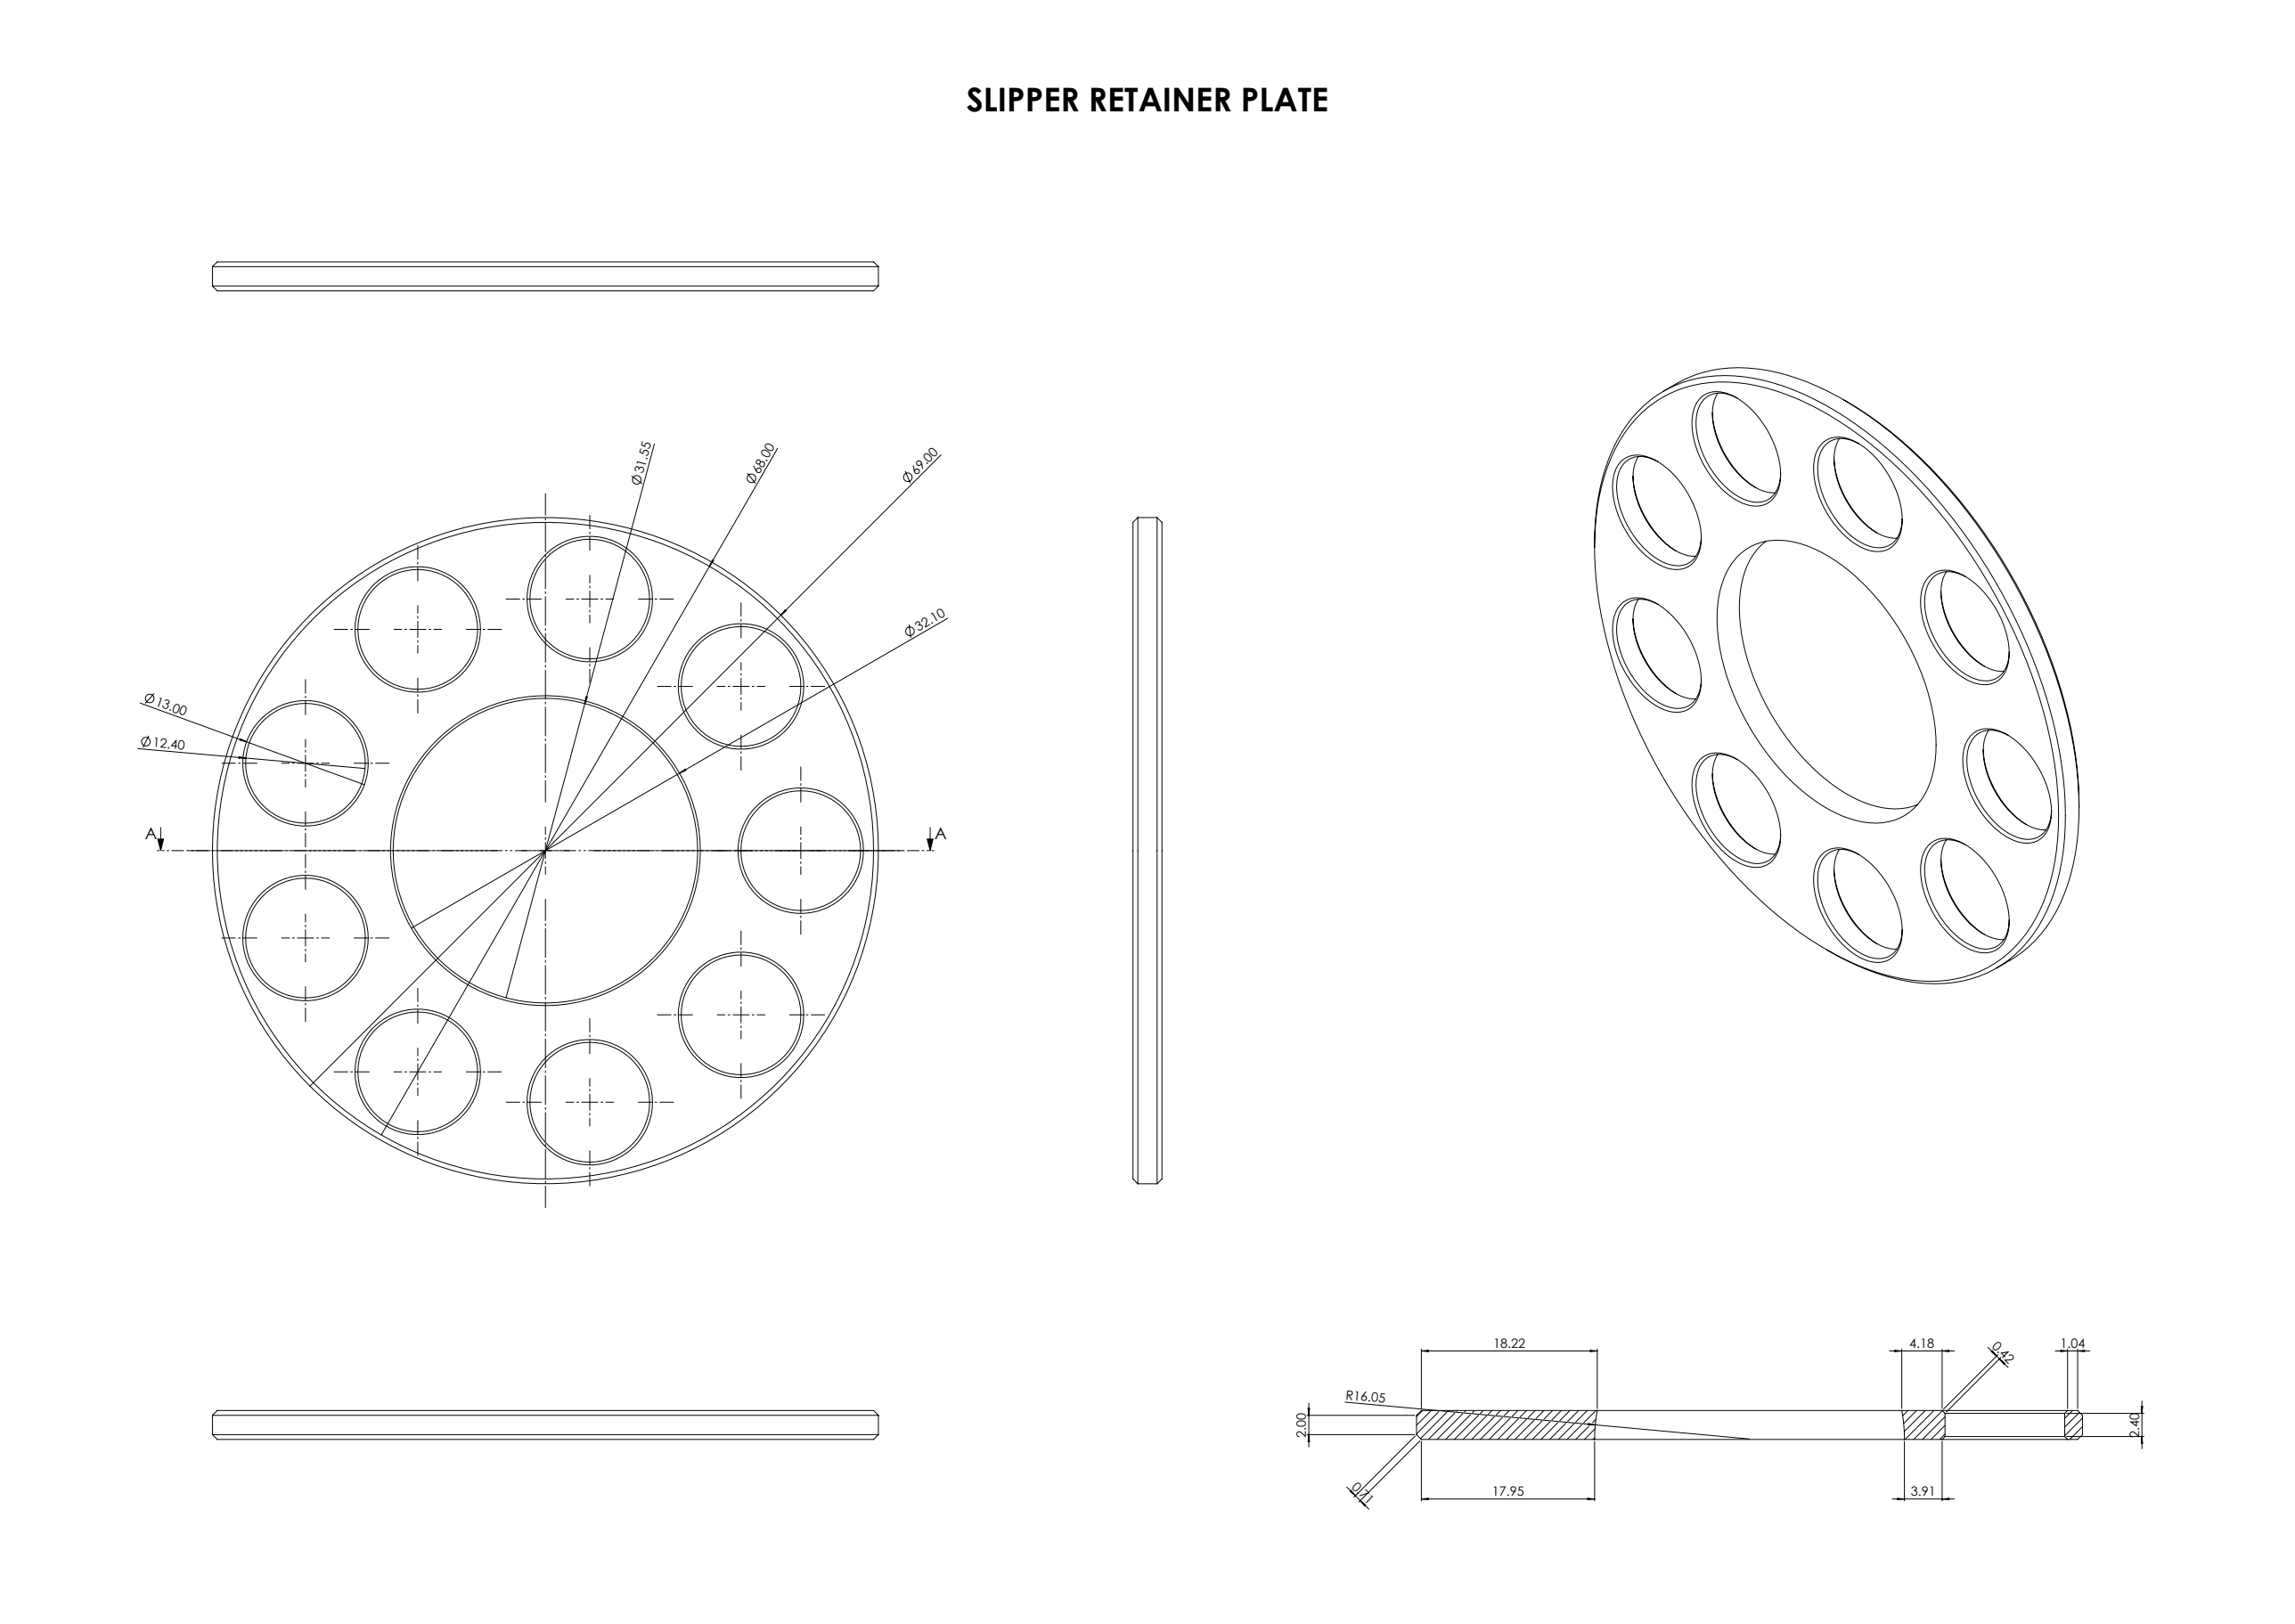
ISO-10303-21;
HEADER;
/* Generated by software containing ST-Developer
 * from STEP Tools, Inc. (www.steptools.com) 
 */

FILE_DESCRIPTION(
/* description */ (''),
/* implementation_level */ '2;1');

FILE_NAME(
/* name */ '08_Slipper_Retainer_Plate.step',
/* time_stamp */ '2026-10-23T00:52:27+05:00',
/* author */ (''),
/* organization */ (''),
/* preprocessor_version */ 'ST-DEVELOPER v20.2',
/* originating_system */ 'Autodesk Translation Framework v15.15.0.0',
/* authorisation */ '');

FILE_SCHEMA (('AUTOMOTIVE_DESIGN { 1 0 10303 214 3 1 1 }'));
ENDSEC;

DATA;
#10=MECHANICAL_DESIGN_GEOMETRIC_PRESENTATION_REPRESENTATION('',(#1548),#59204);
#1508=SHAPE_REPRESENTATION_RELATIONSHIP('SRR','None',#59297,#1528);
#1528=ADVANCED_BREP_SHAPE_REPRESENTATION('',(#1575),#59184);
#1548=STYLED_ITEM('',(#59579),#1575);
#1575=MANIFOLD_SOLID_BREP('Retainer plate',#22804);
#1595=SPHERICAL_SURFACE('',#23116,1.605);
#1599=FACE_BOUND('',#3977,.T.);
#1600=FACE_BOUND('',#3978,.T.);
#1601=FACE_BOUND('',#3979,.T.);
#1602=FACE_BOUND('',#3980,.T.);
#1603=FACE_BOUND('',#3981,.T.);
#1604=FACE_BOUND('',#3982,.T.);
#1605=FACE_BOUND('',#3983,.T.);
#1606=FACE_BOUND('',#3984,.T.);
#1607=FACE_BOUND('',#3985,.T.);
#1608=FACE_BOUND('',#3986,.T.);
#1609=FACE_BOUND('',#3989,.T.);
#1610=FACE_BOUND('',#3990,.T.);
#1611=FACE_BOUND('',#3991,.T.);
#1612=FACE_BOUND('',#3992,.T.);
#1613=FACE_BOUND('',#3993,.T.);
#1614=FACE_BOUND('',#3994,.T.);
#1615=FACE_BOUND('',#3995,.T.);
#1616=FACE_BOUND('',#3996,.T.);
#1617=FACE_BOUND('',#3997,.T.);
#1618=FACE_BOUND('',#3998,.T.);
#1810=PLANE('',#23052);
#1811=PLANE('',#23065);
#2409=CYLINDRICAL_SURFACE('',#23050,0.62);
#2410=CYLINDRICAL_SURFACE('',#23078,0.62);
#2411=CYLINDRICAL_SURFACE('',#23083,0.62);
#2412=CYLINDRICAL_SURFACE('',#23088,0.62);
#2413=CYLINDRICAL_SURFACE('',#23093,0.62);
#2414=CYLINDRICAL_SURFACE('',#23098,0.62);
#2415=CYLINDRICAL_SURFACE('',#23103,0.62);
#2416=CYLINDRICAL_SURFACE('',#23108,0.62);
#2417=CYLINDRICAL_SURFACE('',#23113,0.62);
#2418=CYLINDRICAL_SURFACE('',#23120,3.45);
#2669=FACE_OUTER_BOUND('',#3974,.T.);
#2670=FACE_OUTER_BOUND('',#3975,.T.);
#2671=FACE_OUTER_BOUND('',#3976,.T.);
#2672=FACE_OUTER_BOUND('',#3987,.T.);
#2673=FACE_OUTER_BOUND('',#3988,.T.);
#2674=FACE_OUTER_BOUND('',#3999,.T.);
#2675=FACE_OUTER_BOUND('',#4000,.T.);
#2676=FACE_OUTER_BOUND('',#4001,.T.);
#2677=FACE_OUTER_BOUND('',#4002,.T.);
#2678=FACE_OUTER_BOUND('',#4003,.T.);
#2679=FACE_OUTER_BOUND('',#4004,.T.);
#2680=FACE_OUTER_BOUND('',#4005,.T.);
#2681=FACE_OUTER_BOUND('',#4006,.T.);
#2682=FACE_OUTER_BOUND('',#4007,.T.);
#2683=FACE_OUTER_BOUND('',#4008,.T.);
#2684=FACE_OUTER_BOUND('',#4009,.T.);
#2685=FACE_OUTER_BOUND('',#4010,.T.);
#2686=FACE_OUTER_BOUND('',#4011,.T.);
#2687=FACE_OUTER_BOUND('',#4012,.T.);
#2688=FACE_OUTER_BOUND('',#4013,.T.);
#2689=FACE_OUTER_BOUND('',#4014,.T.);
#2690=FACE_OUTER_BOUND('',#4015,.T.);
#2691=FACE_OUTER_BOUND('',#4016,.T.);
#2692=FACE_OUTER_BOUND('',#4017,.T.);
#2693=FACE_OUTER_BOUND('',#4018,.T.);
#2694=FACE_OUTER_BOUND('',#4019,.T.);
#2695=FACE_OUTER_BOUND('',#4020,.T.);
#2696=FACE_OUTER_BOUND('',#4021,.T.);
#2697=FACE_OUTER_BOUND('',#4022,.T.);
#2698=FACE_OUTER_BOUND('',#4023,.T.);
#2699=FACE_OUTER_BOUND('',#4024,.T.);
#2700=FACE_OUTER_BOUND('',#4025,.T.);
#2701=FACE_OUTER_BOUND('',#4026,.T.);
#3974=EDGE_LOOP('',(#14662,#14663,#14664,#14665));
#3975=EDGE_LOOP('',(#14666,#14667,#14668,#14669));
#3976=EDGE_LOOP('',(#14670));
#3977=EDGE_LOOP('',(#14671));
#3978=EDGE_LOOP('',(#14672));
#3979=EDGE_LOOP('',(#14673));
#3980=EDGE_LOOP('',(#14674));
#3981=EDGE_LOOP('',(#14675));
#3982=EDGE_LOOP('',(#14676));
#3983=EDGE_LOOP('',(#14677));
#3984=EDGE_LOOP('',(#14678));
#3985=EDGE_LOOP('',(#14679));
#3986=EDGE_LOOP('',(#14680));
#3987=EDGE_LOOP('',(#14681,#14682,#14683,#14684));
#3988=EDGE_LOOP('',(#14685));
#3989=EDGE_LOOP('',(#14686));
#3990=EDGE_LOOP('',(#14687));
#3991=EDGE_LOOP('',(#14688));
#3992=EDGE_LOOP('',(#14689));
#3993=EDGE_LOOP('',(#14690));
#3994=EDGE_LOOP('',(#14691));
#3995=EDGE_LOOP('',(#14692));
#3996=EDGE_LOOP('',(#14693));
#3997=EDGE_LOOP('',(#14694));
#3998=EDGE_LOOP('',(#14695));
#3999=EDGE_LOOP('',(#14696,#14697,#14698,#14699));
#4000=EDGE_LOOP('',(#14700,#14701,#14702,#14703));
#4001=EDGE_LOOP('',(#14704,#14705,#14706,#14707));
#4002=EDGE_LOOP('',(#14708,#14709,#14710,#14711));
#4003=EDGE_LOOP('',(#14712,#14713,#14714,#14715));
#4004=EDGE_LOOP('',(#14716,#14717,#14718,#14719));
#4005=EDGE_LOOP('',(#14720,#14721,#14722,#14723));
#4006=EDGE_LOOP('',(#14724,#14725,#14726,#14727));
#4007=EDGE_LOOP('',(#14728,#14729,#14730,#14731));
#4008=EDGE_LOOP('',(#14732,#14733,#14734,#14735));
#4009=EDGE_LOOP('',(#14736,#14737,#14738,#14739));
#4010=EDGE_LOOP('',(#14740,#14741,#14742,#14743));
#4011=EDGE_LOOP('',(#14744,#14745,#14746,#14747));
#4012=EDGE_LOOP('',(#14748,#14749,#14750,#14751));
#4013=EDGE_LOOP('',(#14752,#14753,#14754,#14755));
#4014=EDGE_LOOP('',(#14756,#14757,#14758,#14759));
#4015=EDGE_LOOP('',(#14760,#14761,#14762,#14763));
#4016=EDGE_LOOP('',(#14764,#14765,#14766,#14767));
#4017=EDGE_LOOP('',(#14768,#14769,#14770,#14771));
#4018=EDGE_LOOP('',(#14772,#14773,#14774,#14775));
#4019=EDGE_LOOP('',(#14776,#14777,#14778,#14779));
#4020=EDGE_LOOP('',(#14780,#14781,#14782,#14783));
#4021=EDGE_LOOP('',(#14784,#14785,#14786,#14787));
#4022=EDGE_LOOP('',(#14788,#14789,#14790,#14791));
#4023=EDGE_LOOP('',(#14792,#14793,#14794,#14795));
#4024=EDGE_LOOP('',(#14796,#14797,#14798,#14799));
#4025=EDGE_LOOP('',(#14800,#14801,#14802,#14803));
#4026=EDGE_LOOP('',(#14804,#14805,#14806,#14807));
#5490=LINE('',#30697,#6923);
#5491=LINE('',#30701,#6924);
#5492=LINE('',#30727,#6925);
#5493=LINE('',#30751,#6926);
#5494=LINE('',#30755,#6927);
#5495=LINE('',#30758,#6928);
#5496=LINE('',#30761,#6929);
#5497=LINE('',#30765,#6930);
#5498=LINE('',#30768,#6931);
#5499=LINE('',#30771,#6932);
#5500=LINE('',#30775,#6933);
#5501=LINE('',#30778,#6934);
#5502=LINE('',#30781,#6935);
#5503=LINE('',#30785,#6936);
#5504=LINE('',#30788,#6937);
#5505=LINE('',#30791,#6938);
#5506=LINE('',#30795,#6939);
#5507=LINE('',#30798,#6940);
#5508=LINE('',#30801,#6941);
#5509=LINE('',#30805,#6942);
#5510=LINE('',#30808,#6943);
#5511=LINE('',#30811,#6944);
#5512=LINE('',#30815,#6945);
#5513=LINE('',#30818,#6946);
#5514=LINE('',#30821,#6947);
#5515=LINE('',#30825,#6948);
#5516=LINE('',#30828,#6949);
#5517=LINE('',#30834,#6950);
#5518=LINE('',#30838,#6951);
#5519=LINE('',#30840,#6952);
#6923=VECTOR('',#25124,0.635);
#6924=VECTOR('',#25129,0.62);
#6925=VECTOR('',#25158,0.635);
#6926=VECTOR('',#25183,0.635);
#6927=VECTOR('',#25188,0.62);
#6928=VECTOR('',#25193,0.635);
#6929=VECTOR('',#25196,0.635);
#6930=VECTOR('',#25201,0.62);
#6931=VECTOR('',#25206,0.635);
#6932=VECTOR('',#25209,0.635);
#6933=VECTOR('',#25214,0.62);
#6934=VECTOR('',#25219,0.635);
#6935=VECTOR('',#25222,0.635);
#6936=VECTOR('',#25227,0.62);
#6937=VECTOR('',#25232,0.635);
#6938=VECTOR('',#25235,0.635);
#6939=VECTOR('',#25240,0.62);
#6940=VECTOR('',#25245,0.635);
#6941=VECTOR('',#25248,0.635);
#6942=VECTOR('',#25253,0.62);
#6943=VECTOR('',#25258,0.635);
#6944=VECTOR('',#25261,0.635);
#6945=VECTOR('',#25266,0.62);
#6946=VECTOR('',#25271,0.635);
#6947=VECTOR('',#25274,0.635);
#6948=VECTOR('',#25279,0.62);
#6949=VECTOR('',#25284,0.635);
#6950=VECTOR('',#25293,3.425);
#6951=VECTOR('',#25298,3.45);
#6952=VECTOR('',#25301,3.425);
#8356=CIRCLE('',#23048,0.65);
#8357=CIRCLE('',#23049,0.62);
#8358=CIRCLE('',#23051,0.62);
#8359=CIRCLE('',#23053,3.4);
#8360=CIRCLE('',#23054,0.65);
#8361=CIRCLE('',#23055,0.65);
#8362=CIRCLE('',#23056,0.65);
#8363=CIRCLE('',#23057,0.65);
#8364=CIRCLE('',#23058,1.57765648986083);
#8365=CIRCLE('',#23059,0.65);
#8366=CIRCLE('',#23060,0.65);
#8367=CIRCLE('',#23061,0.65);
#8368=CIRCLE('',#23062,0.65);
#8369=CIRCLE('',#23064,0.65);
#8370=CIRCLE('',#23066,3.4);
#8371=CIRCLE('',#23067,0.65);
#8372=CIRCLE('',#23068,0.65);
#8373=CIRCLE('',#23069,0.65);
#8374=CIRCLE('',#23070,0.65);
#8375=CIRCLE('',#23071,1.60499221181911);
#8376=CIRCLE('',#23072,0.65);
#8377=CIRCLE('',#23073,0.65);
#8378=CIRCLE('',#23074,0.65);
#8379=CIRCLE('',#23075,0.65);
#8380=CIRCLE('',#23077,0.62);
#8381=CIRCLE('',#23079,0.62);
#8382=CIRCLE('',#23082,0.62);
#8383=CIRCLE('',#23084,0.62);
#8384=CIRCLE('',#23087,0.62);
#8385=CIRCLE('',#23089,0.62);
#8386=CIRCLE('',#23092,0.62);
#8387=CIRCLE('',#23094,0.62);
#8388=CIRCLE('',#23097,0.62);
#8389=CIRCLE('',#23099,0.62);
#8390=CIRCLE('',#23102,0.62);
#8391=CIRCLE('',#23104,0.62);
#8392=CIRCLE('',#23107,0.62);
#8393=CIRCLE('',#23109,0.62);
#8394=CIRCLE('',#23112,0.62);
#8395=CIRCLE('',#23114,0.62);
#8396=CIRCLE('',#23117,1.605);
#8397=CIRCLE('',#23119,3.45);
#8398=CIRCLE('',#23121,3.45);
#9192=VERTEX_POINT('',#30694);
#9193=VERTEX_POINT('',#30696);
#9194=VERTEX_POINT('',#30700);
#9195=VERTEX_POINT('',#30704);
#9196=VERTEX_POINT('',#30706);
#9197=VERTEX_POINT('',#30708);
#9198=VERTEX_POINT('',#30710);
#9199=VERTEX_POINT('',#30712);
#9200=VERTEX_POINT('',#30714);
#9201=VERTEX_POINT('',#30716);
#9202=VERTEX_POINT('',#30718);
#9203=VERTEX_POINT('',#30720);
#9204=VERTEX_POINT('',#30722);
#9205=VERTEX_POINT('',#30725);
#9206=VERTEX_POINT('',#30729);
#9207=VERTEX_POINT('',#30731);
#9208=VERTEX_POINT('',#30733);
#9209=VERTEX_POINT('',#30735);
#9210=VERTEX_POINT('',#30737);
#9211=VERTEX_POINT('',#30739);
#9212=VERTEX_POINT('',#30741);
#9213=VERTEX_POINT('',#30743);
#9214=VERTEX_POINT('',#30745);
#9215=VERTEX_POINT('',#30747);
#9216=VERTEX_POINT('',#30750);
#9217=VERTEX_POINT('',#30754);
#9218=VERTEX_POINT('',#30760);
#9219=VERTEX_POINT('',#30764);
#9220=VERTEX_POINT('',#30770);
#9221=VERTEX_POINT('',#30774);
#9222=VERTEX_POINT('',#30780);
#9223=VERTEX_POINT('',#30784);
#9224=VERTEX_POINT('',#30790);
#9225=VERTEX_POINT('',#30794);
#9226=VERTEX_POINT('',#30800);
#9227=VERTEX_POINT('',#30804);
#9228=VERTEX_POINT('',#30810);
#9229=VERTEX_POINT('',#30814);
#9230=VERTEX_POINT('',#30820);
#9231=VERTEX_POINT('',#30824);
#9232=VERTEX_POINT('',#30832);
#9233=VERTEX_POINT('',#30836);
#11335=EDGE_CURVE('',#9192,#9192,#8356,.T.);
#11336=EDGE_CURVE('',#9192,#9193,#5490,.T.);
#11337=EDGE_CURVE('',#9193,#9193,#8357,.T.);
#11338=EDGE_CURVE('',#9193,#9194,#5491,.T.);
#11339=EDGE_CURVE('',#9194,#9194,#8358,.T.);
#11340=EDGE_CURVE('',#9195,#9195,#8359,.T.);
#11341=EDGE_CURVE('',#9196,#9196,#8360,.T.);
#11342=EDGE_CURVE('',#9197,#9197,#8361,.T.);
#11343=EDGE_CURVE('',#9198,#9198,#8362,.T.);
#11344=EDGE_CURVE('',#9199,#9199,#8363,.T.);
#11345=EDGE_CURVE('',#9200,#9200,#8364,.T.);
#11346=EDGE_CURVE('',#9201,#9201,#8365,.T.);
#11347=EDGE_CURVE('',#9202,#9202,#8366,.T.);
#11348=EDGE_CURVE('',#9203,#9203,#8367,.T.);
#11349=EDGE_CURVE('',#9204,#9204,#8368,.T.);
#11350=EDGE_CURVE('',#9205,#9205,#8369,.T.);
#11351=EDGE_CURVE('',#9205,#9194,#5492,.T.);
#11352=EDGE_CURVE('',#9206,#9206,#8370,.T.);
#11353=EDGE_CURVE('',#9207,#9207,#8371,.T.);
#11354=EDGE_CURVE('',#9208,#9208,#8372,.T.);
#11355=EDGE_CURVE('',#9209,#9209,#8373,.T.);
#11356=EDGE_CURVE('',#9210,#9210,#8374,.T.);
#11357=EDGE_CURVE('',#9211,#9211,#8375,.T.);
#11358=EDGE_CURVE('',#9212,#9212,#8376,.T.);
#11359=EDGE_CURVE('',#9213,#9213,#8377,.T.);
#11360=EDGE_CURVE('',#9214,#9214,#8378,.T.);
#11361=EDGE_CURVE('',#9215,#9215,#8379,.T.);
#11362=EDGE_CURVE('',#9196,#9216,#5493,.T.);
#11363=EDGE_CURVE('',#9216,#9216,#8380,.T.);
#11364=EDGE_CURVE('',#9216,#9217,#5494,.T.);
#11365=EDGE_CURVE('',#9217,#9217,#8381,.T.);
#11366=EDGE_CURVE('',#9207,#9217,#5495,.T.);
#11367=EDGE_CURVE('',#9204,#9218,#5496,.T.);
#11368=EDGE_CURVE('',#9218,#9218,#8382,.T.);
#11369=EDGE_CURVE('',#9218,#9219,#5497,.T.);
#11370=EDGE_CURVE('',#9219,#9219,#8383,.T.);
#11371=EDGE_CURVE('',#9215,#9219,#5498,.T.);
#11372=EDGE_CURVE('',#9197,#9220,#5499,.T.);
#11373=EDGE_CURVE('',#9220,#9220,#8384,.T.);
#11374=EDGE_CURVE('',#9220,#9221,#5500,.T.);
#11375=EDGE_CURVE('',#9221,#9221,#8385,.T.);
#11376=EDGE_CURVE('',#9208,#9221,#5501,.T.);
#11377=EDGE_CURVE('',#9203,#9222,#5502,.T.);
#11378=EDGE_CURVE('',#9222,#9222,#8386,.T.);
#11379=EDGE_CURVE('',#9222,#9223,#5503,.T.);
#11380=EDGE_CURVE('',#9223,#9223,#8387,.T.);
#11381=EDGE_CURVE('',#9214,#9223,#5504,.T.);
#11382=EDGE_CURVE('',#9198,#9224,#5505,.T.);
#11383=EDGE_CURVE('',#9224,#9224,#8388,.T.);
#11384=EDGE_CURVE('',#9224,#9225,#5506,.T.);
#11385=EDGE_CURVE('',#9225,#9225,#8389,.T.);
#11386=EDGE_CURVE('',#9209,#9225,#5507,.T.);
#11387=EDGE_CURVE('',#9202,#9226,#5508,.T.);
#11388=EDGE_CURVE('',#9226,#9226,#8390,.T.);
#11389=EDGE_CURVE('',#9226,#9227,#5509,.T.);
#11390=EDGE_CURVE('',#9227,#9227,#8391,.T.);
#11391=EDGE_CURVE('',#9213,#9227,#5510,.T.);
#11392=EDGE_CURVE('',#9199,#9228,#5511,.T.);
#11393=EDGE_CURVE('',#9228,#9228,#8392,.T.);
#11394=EDGE_CURVE('',#9228,#9229,#5512,.T.);
#11395=EDGE_CURVE('',#9229,#9229,#8393,.T.);
#11396=EDGE_CURVE('',#9210,#9229,#5513,.T.);
#11397=EDGE_CURVE('',#9201,#9230,#5514,.T.);
#11398=EDGE_CURVE('',#9230,#9230,#8394,.T.);
#11399=EDGE_CURVE('',#9230,#9231,#5515,.T.);
#11400=EDGE_CURVE('',#9231,#9231,#8395,.T.);
#11401=EDGE_CURVE('',#9212,#9231,#5516,.T.);
#11402=EDGE_CURVE('',#9211,#9200,#8396,.T.);
#11403=EDGE_CURVE('',#9232,#9232,#8397,.T.);
#11404=EDGE_CURVE('',#9232,#9195,#5517,.T.);
#11405=EDGE_CURVE('',#9233,#9233,#8398,.T.);
#11406=EDGE_CURVE('',#9233,#9232,#5518,.T.);
#11407=EDGE_CURVE('',#9206,#9233,#5519,.T.);
#14662=ORIENTED_EDGE('',*,*,#11335,.T.);
#14663=ORIENTED_EDGE('',*,*,#11336,.T.);
#14664=ORIENTED_EDGE('',*,*,#11337,.T.);
#14665=ORIENTED_EDGE('',*,*,#11336,.F.);
#14666=ORIENTED_EDGE('',*,*,#11337,.F.);
#14667=ORIENTED_EDGE('',*,*,#11338,.T.);
#14668=ORIENTED_EDGE('',*,*,#11339,.F.);
#14669=ORIENTED_EDGE('',*,*,#11338,.F.);
#14670=ORIENTED_EDGE('',*,*,#11340,.F.);
#14671=ORIENTED_EDGE('',*,*,#11341,.F.);
#14672=ORIENTED_EDGE('',*,*,#11342,.F.);
#14673=ORIENTED_EDGE('',*,*,#11343,.F.);
#14674=ORIENTED_EDGE('',*,*,#11344,.F.);
#14675=ORIENTED_EDGE('',*,*,#11345,.T.);
#14676=ORIENTED_EDGE('',*,*,#11346,.F.);
#14677=ORIENTED_EDGE('',*,*,#11347,.F.);
#14678=ORIENTED_EDGE('',*,*,#11348,.F.);
#14679=ORIENTED_EDGE('',*,*,#11349,.F.);
#14680=ORIENTED_EDGE('',*,*,#11335,.F.);
#14681=ORIENTED_EDGE('',*,*,#11350,.T.);
#14682=ORIENTED_EDGE('',*,*,#11351,.T.);
#14683=ORIENTED_EDGE('',*,*,#11339,.T.);
#14684=ORIENTED_EDGE('',*,*,#11351,.F.);
#14685=ORIENTED_EDGE('',*,*,#11352,.T.);
#14686=ORIENTED_EDGE('',*,*,#11353,.F.);
#14687=ORIENTED_EDGE('',*,*,#11354,.F.);
#14688=ORIENTED_EDGE('',*,*,#11355,.F.);
#14689=ORIENTED_EDGE('',*,*,#11356,.F.);
#14690=ORIENTED_EDGE('',*,*,#11357,.F.);
#14691=ORIENTED_EDGE('',*,*,#11358,.F.);
#14692=ORIENTED_EDGE('',*,*,#11359,.F.);
#14693=ORIENTED_EDGE('',*,*,#11360,.F.);
#14694=ORIENTED_EDGE('',*,*,#11361,.F.);
#14695=ORIENTED_EDGE('',*,*,#11350,.F.);
#14696=ORIENTED_EDGE('',*,*,#11341,.T.);
#14697=ORIENTED_EDGE('',*,*,#11362,.T.);
#14698=ORIENTED_EDGE('',*,*,#11363,.T.);
#14699=ORIENTED_EDGE('',*,*,#11362,.F.);
#14700=ORIENTED_EDGE('',*,*,#11363,.F.);
#14701=ORIENTED_EDGE('',*,*,#11364,.T.);
#14702=ORIENTED_EDGE('',*,*,#11365,.F.);
#14703=ORIENTED_EDGE('',*,*,#11364,.F.);
#14704=ORIENTED_EDGE('',*,*,#11353,.T.);
#14705=ORIENTED_EDGE('',*,*,#11366,.T.);
#14706=ORIENTED_EDGE('',*,*,#11365,.T.);
#14707=ORIENTED_EDGE('',*,*,#11366,.F.);
#14708=ORIENTED_EDGE('',*,*,#11349,.T.);
#14709=ORIENTED_EDGE('',*,*,#11367,.T.);
#14710=ORIENTED_EDGE('',*,*,#11368,.T.);
#14711=ORIENTED_EDGE('',*,*,#11367,.F.);
#14712=ORIENTED_EDGE('',*,*,#11368,.F.);
#14713=ORIENTED_EDGE('',*,*,#11369,.T.);
#14714=ORIENTED_EDGE('',*,*,#11370,.F.);
#14715=ORIENTED_EDGE('',*,*,#11369,.F.);
#14716=ORIENTED_EDGE('',*,*,#11361,.T.);
#14717=ORIENTED_EDGE('',*,*,#11371,.T.);
#14718=ORIENTED_EDGE('',*,*,#11370,.T.);
#14719=ORIENTED_EDGE('',*,*,#11371,.F.);
#14720=ORIENTED_EDGE('',*,*,#11342,.T.);
#14721=ORIENTED_EDGE('',*,*,#11372,.T.);
#14722=ORIENTED_EDGE('',*,*,#11373,.T.);
#14723=ORIENTED_EDGE('',*,*,#11372,.F.);
#14724=ORIENTED_EDGE('',*,*,#11373,.F.);
#14725=ORIENTED_EDGE('',*,*,#11374,.T.);
#14726=ORIENTED_EDGE('',*,*,#11375,.F.);
#14727=ORIENTED_EDGE('',*,*,#11374,.F.);
#14728=ORIENTED_EDGE('',*,*,#11354,.T.);
#14729=ORIENTED_EDGE('',*,*,#11376,.T.);
#14730=ORIENTED_EDGE('',*,*,#11375,.T.);
#14731=ORIENTED_EDGE('',*,*,#11376,.F.);
#14732=ORIENTED_EDGE('',*,*,#11348,.T.);
#14733=ORIENTED_EDGE('',*,*,#11377,.T.);
#14734=ORIENTED_EDGE('',*,*,#11378,.T.);
#14735=ORIENTED_EDGE('',*,*,#11377,.F.);
#14736=ORIENTED_EDGE('',*,*,#11378,.F.);
#14737=ORIENTED_EDGE('',*,*,#11379,.T.);
#14738=ORIENTED_EDGE('',*,*,#11380,.F.);
#14739=ORIENTED_EDGE('',*,*,#11379,.F.);
#14740=ORIENTED_EDGE('',*,*,#11360,.T.);
#14741=ORIENTED_EDGE('',*,*,#11381,.T.);
#14742=ORIENTED_EDGE('',*,*,#11380,.T.);
#14743=ORIENTED_EDGE('',*,*,#11381,.F.);
#14744=ORIENTED_EDGE('',*,*,#11343,.T.);
#14745=ORIENTED_EDGE('',*,*,#11382,.T.);
#14746=ORIENTED_EDGE('',*,*,#11383,.T.);
#14747=ORIENTED_EDGE('',*,*,#11382,.F.);
#14748=ORIENTED_EDGE('',*,*,#11383,.F.);
#14749=ORIENTED_EDGE('',*,*,#11384,.T.);
#14750=ORIENTED_EDGE('',*,*,#11385,.F.);
#14751=ORIENTED_EDGE('',*,*,#11384,.F.);
#14752=ORIENTED_EDGE('',*,*,#11355,.T.);
#14753=ORIENTED_EDGE('',*,*,#11386,.T.);
#14754=ORIENTED_EDGE('',*,*,#11385,.T.);
#14755=ORIENTED_EDGE('',*,*,#11386,.F.);
#14756=ORIENTED_EDGE('',*,*,#11347,.T.);
#14757=ORIENTED_EDGE('',*,*,#11387,.T.);
#14758=ORIENTED_EDGE('',*,*,#11388,.T.);
#14759=ORIENTED_EDGE('',*,*,#11387,.F.);
#14760=ORIENTED_EDGE('',*,*,#11388,.F.);
#14761=ORIENTED_EDGE('',*,*,#11389,.T.);
#14762=ORIENTED_EDGE('',*,*,#11390,.F.);
#14763=ORIENTED_EDGE('',*,*,#11389,.F.);
#14764=ORIENTED_EDGE('',*,*,#11359,.T.);
#14765=ORIENTED_EDGE('',*,*,#11391,.T.);
#14766=ORIENTED_EDGE('',*,*,#11390,.T.);
#14767=ORIENTED_EDGE('',*,*,#11391,.F.);
#14768=ORIENTED_EDGE('',*,*,#11344,.T.);
#14769=ORIENTED_EDGE('',*,*,#11392,.T.);
#14770=ORIENTED_EDGE('',*,*,#11393,.T.);
#14771=ORIENTED_EDGE('',*,*,#11392,.F.);
#14772=ORIENTED_EDGE('',*,*,#11393,.F.);
#14773=ORIENTED_EDGE('',*,*,#11394,.T.);
#14774=ORIENTED_EDGE('',*,*,#11395,.F.);
#14775=ORIENTED_EDGE('',*,*,#11394,.F.);
#14776=ORIENTED_EDGE('',*,*,#11356,.T.);
#14777=ORIENTED_EDGE('',*,*,#11396,.T.);
#14778=ORIENTED_EDGE('',*,*,#11395,.T.);
#14779=ORIENTED_EDGE('',*,*,#11396,.F.);
#14780=ORIENTED_EDGE('',*,*,#11346,.T.);
#14781=ORIENTED_EDGE('',*,*,#11397,.T.);
#14782=ORIENTED_EDGE('',*,*,#11398,.T.);
#14783=ORIENTED_EDGE('',*,*,#11397,.F.);
#14784=ORIENTED_EDGE('',*,*,#11398,.F.);
#14785=ORIENTED_EDGE('',*,*,#11399,.T.);
#14786=ORIENTED_EDGE('',*,*,#11400,.F.);
#14787=ORIENTED_EDGE('',*,*,#11399,.F.);
#14788=ORIENTED_EDGE('',*,*,#11358,.T.);
#14789=ORIENTED_EDGE('',*,*,#11401,.T.);
#14790=ORIENTED_EDGE('',*,*,#11400,.T.);
#14791=ORIENTED_EDGE('',*,*,#11401,.F.);
#14792=ORIENTED_EDGE('',*,*,#11357,.T.);
#14793=ORIENTED_EDGE('',*,*,#11402,.T.);
#14794=ORIENTED_EDGE('',*,*,#11345,.F.);
#14795=ORIENTED_EDGE('',*,*,#11402,.F.);
#14796=ORIENTED_EDGE('',*,*,#11403,.F.);
#14797=ORIENTED_EDGE('',*,*,#11404,.T.);
#14798=ORIENTED_EDGE('',*,*,#11340,.T.);
#14799=ORIENTED_EDGE('',*,*,#11404,.F.);
#14800=ORIENTED_EDGE('',*,*,#11405,.F.);
#14801=ORIENTED_EDGE('',*,*,#11406,.T.);
#14802=ORIENTED_EDGE('',*,*,#11403,.T.);
#14803=ORIENTED_EDGE('',*,*,#11406,.F.);
#14804=ORIENTED_EDGE('',*,*,#11352,.F.);
#14805=ORIENTED_EDGE('',*,*,#11407,.T.);
#14806=ORIENTED_EDGE('',*,*,#11405,.T.);
#14807=ORIENTED_EDGE('',*,*,#11407,.F.);
#21316=CONICAL_SURFACE('',#23047,0.635,0.785398163397444);
#21317=CONICAL_SURFACE('',#23063,0.635,0.785398163397445);
#21318=CONICAL_SURFACE('',#23076,0.635,0.785398163397448);
#21319=CONICAL_SURFACE('',#23080,0.635,0.785398163397448);
#21320=CONICAL_SURFACE('',#23081,0.635,0.785398163397448);
#21321=CONICAL_SURFACE('',#23085,0.635,0.785398163397448);
#21322=CONICAL_SURFACE('',#23086,0.635,0.785398163397444);
#21323=CONICAL_SURFACE('',#23090,0.635,0.785398163397445);
#21324=CONICAL_SURFACE('',#23091,0.635,0.785398163397444);
#21325=CONICAL_SURFACE('',#23095,0.635,0.785398163397445);
#21326=CONICAL_SURFACE('',#23096,0.635,0.785398163397448);
#21327=CONICAL_SURFACE('',#23100,0.635,0.785398163397448);
#21328=CONICAL_SURFACE('',#23101,0.635,0.785398163397448);
#21329=CONICAL_SURFACE('',#23105,0.635,0.785398163397448);
#21330=CONICAL_SURFACE('',#23106,0.635,0.785398163397448);
#21331=CONICAL_SURFACE('',#23110,0.635,0.785398163397448);
#21332=CONICAL_SURFACE('',#23111,0.635,0.785398163397448);
#21333=CONICAL_SURFACE('',#23115,0.635,0.785398163397448);
#21334=CONICAL_SURFACE('',#23118,3.425,0.785398163397451);
#21335=CONICAL_SURFACE('',#23122,3.425,0.785398163397451);
#21499=ADVANCED_FACE('',(#2669),#21316,.F.);
#21500=ADVANCED_FACE('',(#2670),#2409,.F.);
#21501=ADVANCED_FACE('',(#2671,#1599,#1600,#1601,#1602,#1603,#1604,#1605,
#1606,#1607,#1608),#1810,.T.);
#21502=ADVANCED_FACE('',(#2672),#21317,.F.);
#21503=ADVANCED_FACE('',(#2673,#1609,#1610,#1611,#1612,#1613,#1614,#1615,
#1616,#1617,#1618),#1811,.T.);
#21504=ADVANCED_FACE('',(#2674),#21318,.F.);
#21505=ADVANCED_FACE('',(#2675),#2410,.F.);
#21506=ADVANCED_FACE('',(#2676),#21319,.F.);
#21507=ADVANCED_FACE('',(#2677),#21320,.F.);
#21508=ADVANCED_FACE('',(#2678),#2411,.F.);
#21509=ADVANCED_FACE('',(#2679),#21321,.F.);
#21510=ADVANCED_FACE('',(#2680),#21322,.F.);
#21511=ADVANCED_FACE('',(#2681),#2412,.F.);
#21512=ADVANCED_FACE('',(#2682),#21323,.F.);
#21513=ADVANCED_FACE('',(#2683),#21324,.F.);
#21514=ADVANCED_FACE('',(#2684),#2413,.F.);
#21515=ADVANCED_FACE('',(#2685),#21325,.F.);
#21516=ADVANCED_FACE('',(#2686),#21326,.F.);
#21517=ADVANCED_FACE('',(#2687),#2414,.F.);
#21518=ADVANCED_FACE('',(#2688),#21327,.F.);
#21519=ADVANCED_FACE('',(#2689),#21328,.F.);
#21520=ADVANCED_FACE('',(#2690),#2415,.F.);
#21521=ADVANCED_FACE('',(#2691),#21329,.F.);
#21522=ADVANCED_FACE('',(#2692),#21330,.F.);
#21523=ADVANCED_FACE('',(#2693),#2416,.F.);
#21524=ADVANCED_FACE('',(#2694),#21331,.F.);
#21525=ADVANCED_FACE('',(#2695),#21332,.F.);
#21526=ADVANCED_FACE('',(#2696),#2417,.F.);
#21527=ADVANCED_FACE('',(#2697),#21333,.F.);
#21528=ADVANCED_FACE('',(#2698),#1595,.F.);
#21529=ADVANCED_FACE('',(#2699),#21334,.T.);
#21530=ADVANCED_FACE('',(#2700),#2418,.T.);
#21531=ADVANCED_FACE('',(#2701),#21335,.T.);
#22804=CLOSED_SHELL('',(#21499,#21500,#21501,#21502,#21503,#21504,#21505,
#21506,#21507,#21508,#21509,#21510,#21511,#21512,#21513,#21514,#21515,#21516,
#21517,#21518,#21519,#21520,#21521,#21522,#21523,#21524,#21525,#21526,#21527,
#21528,#21529,#21530,#21531));
#23046=AXIS2_PLACEMENT_3D('',#30692,#25118,#25119);
#23047=AXIS2_PLACEMENT_3D('',#30693,#25120,#25121);
#23048=AXIS2_PLACEMENT_3D('',#30695,#25122,#25123);
#23049=AXIS2_PLACEMENT_3D('',#30698,#25125,#25126);
#23050=AXIS2_PLACEMENT_3D('',#30699,#25127,#25128);
#23051=AXIS2_PLACEMENT_3D('',#30702,#25130,#25131);
#23052=AXIS2_PLACEMENT_3D('',#30703,#25132,#25133);
#23053=AXIS2_PLACEMENT_3D('',#30705,#25134,#25135);
#23054=AXIS2_PLACEMENT_3D('',#30707,#25136,#25137);
#23055=AXIS2_PLACEMENT_3D('',#30709,#25138,#25139);
#23056=AXIS2_PLACEMENT_3D('',#30711,#25140,#25141);
#23057=AXIS2_PLACEMENT_3D('',#30713,#25142,#25143);
#23058=AXIS2_PLACEMENT_3D('',#30715,#25144,#25145);
#23059=AXIS2_PLACEMENT_3D('',#30717,#25146,#25147);
#23060=AXIS2_PLACEMENT_3D('',#30719,#25148,#25149);
#23061=AXIS2_PLACEMENT_3D('',#30721,#25150,#25151);
#23062=AXIS2_PLACEMENT_3D('',#30723,#25152,#25153);
#23063=AXIS2_PLACEMENT_3D('',#30724,#25154,#25155);
#23064=AXIS2_PLACEMENT_3D('',#30726,#25156,#25157);
#23065=AXIS2_PLACEMENT_3D('',#30728,#25159,#25160);
#23066=AXIS2_PLACEMENT_3D('',#30730,#25161,#25162);
#23067=AXIS2_PLACEMENT_3D('',#30732,#25163,#25164);
#23068=AXIS2_PLACEMENT_3D('',#30734,#25165,#25166);
#23069=AXIS2_PLACEMENT_3D('',#30736,#25167,#25168);
#23070=AXIS2_PLACEMENT_3D('',#30738,#25169,#25170);
#23071=AXIS2_PLACEMENT_3D('',#30740,#25171,#25172);
#23072=AXIS2_PLACEMENT_3D('',#30742,#25173,#25174);
#23073=AXIS2_PLACEMENT_3D('',#30744,#25175,#25176);
#23074=AXIS2_PLACEMENT_3D('',#30746,#25177,#25178);
#23075=AXIS2_PLACEMENT_3D('',#30748,#25179,#25180);
#23076=AXIS2_PLACEMENT_3D('',#30749,#25181,#25182);
#23077=AXIS2_PLACEMENT_3D('',#30752,#25184,#25185);
#23078=AXIS2_PLACEMENT_3D('',#30753,#25186,#25187);
#23079=AXIS2_PLACEMENT_3D('',#30756,#25189,#25190);
#23080=AXIS2_PLACEMENT_3D('',#30757,#25191,#25192);
#23081=AXIS2_PLACEMENT_3D('',#30759,#25194,#25195);
#23082=AXIS2_PLACEMENT_3D('',#30762,#25197,#25198);
#23083=AXIS2_PLACEMENT_3D('',#30763,#25199,#25200);
#23084=AXIS2_PLACEMENT_3D('',#30766,#25202,#25203);
#23085=AXIS2_PLACEMENT_3D('',#30767,#25204,#25205);
#23086=AXIS2_PLACEMENT_3D('',#30769,#25207,#25208);
#23087=AXIS2_PLACEMENT_3D('',#30772,#25210,#25211);
#23088=AXIS2_PLACEMENT_3D('',#30773,#25212,#25213);
#23089=AXIS2_PLACEMENT_3D('',#30776,#25215,#25216);
#23090=AXIS2_PLACEMENT_3D('',#30777,#25217,#25218);
#23091=AXIS2_PLACEMENT_3D('',#30779,#25220,#25221);
#23092=AXIS2_PLACEMENT_3D('',#30782,#25223,#25224);
#23093=AXIS2_PLACEMENT_3D('',#30783,#25225,#25226);
#23094=AXIS2_PLACEMENT_3D('',#30786,#25228,#25229);
#23095=AXIS2_PLACEMENT_3D('',#30787,#25230,#25231);
#23096=AXIS2_PLACEMENT_3D('',#30789,#25233,#25234);
#23097=AXIS2_PLACEMENT_3D('',#30792,#25236,#25237);
#23098=AXIS2_PLACEMENT_3D('',#30793,#25238,#25239);
#23099=AXIS2_PLACEMENT_3D('',#30796,#25241,#25242);
#23100=AXIS2_PLACEMENT_3D('',#30797,#25243,#25244);
#23101=AXIS2_PLACEMENT_3D('',#30799,#25246,#25247);
#23102=AXIS2_PLACEMENT_3D('',#30802,#25249,#25250);
#23103=AXIS2_PLACEMENT_3D('',#30803,#25251,#25252);
#23104=AXIS2_PLACEMENT_3D('',#30806,#25254,#25255);
#23105=AXIS2_PLACEMENT_3D('',#30807,#25256,#25257);
#23106=AXIS2_PLACEMENT_3D('',#30809,#25259,#25260);
#23107=AXIS2_PLACEMENT_3D('',#30812,#25262,#25263);
#23108=AXIS2_PLACEMENT_3D('',#30813,#25264,#25265);
#23109=AXIS2_PLACEMENT_3D('',#30816,#25267,#25268);
#23110=AXIS2_PLACEMENT_3D('',#30817,#25269,#25270);
#23111=AXIS2_PLACEMENT_3D('',#30819,#25272,#25273);
#23112=AXIS2_PLACEMENT_3D('',#30822,#25275,#25276);
#23113=AXIS2_PLACEMENT_3D('',#30823,#25277,#25278);
#23114=AXIS2_PLACEMENT_3D('',#30826,#25280,#25281);
#23115=AXIS2_PLACEMENT_3D('',#30827,#25282,#25283);
#23116=AXIS2_PLACEMENT_3D('',#30829,#25285,#25286);
#23117=AXIS2_PLACEMENT_3D('',#30830,#25287,#25288);
#23118=AXIS2_PLACEMENT_3D('',#30831,#25289,#25290);
#23119=AXIS2_PLACEMENT_3D('',#30833,#25291,#25292);
#23120=AXIS2_PLACEMENT_3D('',#30835,#25294,#25295);
#23121=AXIS2_PLACEMENT_3D('',#30837,#25296,#25297);
#23122=AXIS2_PLACEMENT_3D('',#30839,#25299,#25300);
#25118=DIRECTION('axis',(0.,0.,1.));
#25119=DIRECTION('refdir',(1.,0.,0.));
#25120=DIRECTION('center_axis',(0.,0.,-1.));
#25121=DIRECTION('ref_axis',(1.,0.,0.));
#25122=DIRECTION('center_axis',(0.,0.,-1.));
#25123=DIRECTION('ref_axis',(1.,0.,0.));
#25124=DIRECTION('',(0.707106781186545,-8.6595605623549E-17,0.70710678118655));
#25125=DIRECTION('center_axis',(0.,0.,1.));
#25126=DIRECTION('ref_axis',(1.,0.,0.));
#25127=DIRECTION('center_axis',(0.,0.,1.));
#25128=DIRECTION('ref_axis',(1.,0.,0.));
#25129=DIRECTION('',(0.,0.,1.));
#25130=DIRECTION('center_axis',(0.,0.,-1.));
#25131=DIRECTION('ref_axis',(1.,0.,0.));
#25132=DIRECTION('center_axis',(0.,0.,-1.));
#25133=DIRECTION('ref_axis',(-1.,0.,0.));
#25134=DIRECTION('center_axis',(0.,0.,1.));
#25135=DIRECTION('ref_axis',(1.,0.,0.));
#25136=DIRECTION('center_axis',(0.,0.,-1.));
#25137=DIRECTION('ref_axis',(1.,0.,0.));
#25138=DIRECTION('center_axis',(0.,0.,-1.));
#25139=DIRECTION('ref_axis',(1.,0.,0.));
#25140=DIRECTION('center_axis',(0.,0.,-1.));
#25141=DIRECTION('ref_axis',(1.,0.,0.));
#25142=DIRECTION('center_axis',(0.,0.,-1.));
#25143=DIRECTION('ref_axis',(1.,0.,0.));
#25144=DIRECTION('center_axis',(0.,0.,1.));
#25145=DIRECTION('ref_axis',(1.,0.,0.));
#25146=DIRECTION('center_axis',(0.,0.,-1.));
#25147=DIRECTION('ref_axis',(1.,0.,0.));
#25148=DIRECTION('center_axis',(0.,0.,-1.));
#25149=DIRECTION('ref_axis',(1.,0.,0.));
#25150=DIRECTION('center_axis',(0.,0.,-1.));
#25151=DIRECTION('ref_axis',(1.,0.,0.));
#25152=DIRECTION('center_axis',(0.,0.,-1.));
#25153=DIRECTION('ref_axis',(1.,0.,0.));
#25154=DIRECTION('center_axis',(0.,0.,1.));
#25155=DIRECTION('ref_axis',(1.,0.,0.));
#25156=DIRECTION('center_axis',(0.,0.,1.));
#25157=DIRECTION('ref_axis',(1.,0.,0.));
#25158=DIRECTION('',(0.707106781186545,8.6595605623549E-17,-0.70710678118655));
#25159=DIRECTION('center_axis',(0.,0.,1.));
#25160=DIRECTION('ref_axis',(1.,0.,0.));
#25161=DIRECTION('center_axis',(0.,0.,1.));
#25162=DIRECTION('ref_axis',(1.,0.,0.));
#25163=DIRECTION('center_axis',(0.,0.,1.));
#25164=DIRECTION('ref_axis',(1.,0.,0.));
#25165=DIRECTION('center_axis',(0.,0.,1.));
#25166=DIRECTION('ref_axis',(1.,0.,0.));
#25167=DIRECTION('center_axis',(0.,0.,1.));
#25168=DIRECTION('ref_axis',(1.,0.,0.));
#25169=DIRECTION('center_axis',(0.,0.,1.));
#25170=DIRECTION('ref_axis',(1.,0.,0.));
#25171=DIRECTION('center_axis',(0.,0.,1.));
#25172=DIRECTION('ref_axis',(1.,0.,0.));
#25173=DIRECTION('center_axis',(0.,0.,1.));
#25174=DIRECTION('ref_axis',(1.,0.,0.));
#25175=DIRECTION('center_axis',(0.,0.,1.));
#25176=DIRECTION('ref_axis',(1.,0.,0.));
#25177=DIRECTION('center_axis',(0.,0.,1.));
#25178=DIRECTION('ref_axis',(1.,0.,0.));
#25179=DIRECTION('center_axis',(0.,0.,1.));
#25180=DIRECTION('ref_axis',(1.,0.,0.));
#25181=DIRECTION('center_axis',(0.,0.,-1.));
#25182=DIRECTION('ref_axis',(1.,0.,0.));
#25183=DIRECTION('',(0.707106781186548,-8.65956056235493E-17,0.707106781186548));
#25184=DIRECTION('center_axis',(0.,0.,1.));
#25185=DIRECTION('ref_axis',(1.,0.,0.));
#25186=DIRECTION('center_axis',(0.,0.,1.));
#25187=DIRECTION('ref_axis',(1.,0.,0.));
#25188=DIRECTION('',(0.,0.,1.));
#25189=DIRECTION('center_axis',(0.,0.,-1.));
#25190=DIRECTION('ref_axis',(1.,0.,0.));
#25191=DIRECTION('center_axis',(0.,0.,1.));
#25192=DIRECTION('ref_axis',(1.,0.,0.));
#25193=DIRECTION('',(0.707106781186548,8.65956056235493E-17,-0.707106781186547));
#25194=DIRECTION('center_axis',(0.,0.,-1.));
#25195=DIRECTION('ref_axis',(1.,0.,0.));
#25196=DIRECTION('',(0.707106781186547,-8.65956056235493E-17,0.707106781186547));
#25197=DIRECTION('center_axis',(0.,0.,1.));
#25198=DIRECTION('ref_axis',(1.,0.,0.));
#25199=DIRECTION('center_axis',(0.,0.,1.));
#25200=DIRECTION('ref_axis',(1.,0.,0.));
#25201=DIRECTION('',(0.,0.,1.));
#25202=DIRECTION('center_axis',(0.,0.,-1.));
#25203=DIRECTION('ref_axis',(1.,0.,0.));
#25204=DIRECTION('center_axis',(0.,0.,1.));
#25205=DIRECTION('ref_axis',(1.,0.,0.));
#25206=DIRECTION('',(0.707106781186548,8.65956056235493E-17,-0.707106781186547));
#25207=DIRECTION('center_axis',(0.,0.,-1.));
#25208=DIRECTION('ref_axis',(1.,0.,0.));
#25209=DIRECTION('',(0.707106781186545,-8.6595605623549E-17,0.70710678118655));
#25210=DIRECTION('center_axis',(0.,0.,1.));
#25211=DIRECTION('ref_axis',(1.,0.,0.));
#25212=DIRECTION('center_axis',(0.,0.,1.));
#25213=DIRECTION('ref_axis',(1.,0.,0.));
#25214=DIRECTION('',(0.,0.,1.));
#25215=DIRECTION('center_axis',(0.,0.,-1.));
#25216=DIRECTION('ref_axis',(1.,0.,0.));
#25217=DIRECTION('center_axis',(0.,0.,1.));
#25218=DIRECTION('ref_axis',(1.,0.,0.));
#25219=DIRECTION('',(0.707106781186545,8.6595605623549E-17,-0.70710678118655));
#25220=DIRECTION('center_axis',(0.,0.,-1.));
#25221=DIRECTION('ref_axis',(1.,0.,0.));
#25222=DIRECTION('',(0.707106781186545,-8.6595605623549E-17,0.70710678118655));
#25223=DIRECTION('center_axis',(0.,0.,1.));
#25224=DIRECTION('ref_axis',(1.,0.,0.));
#25225=DIRECTION('center_axis',(0.,0.,1.));
#25226=DIRECTION('ref_axis',(1.,0.,0.));
#25227=DIRECTION('',(0.,0.,1.));
#25228=DIRECTION('center_axis',(0.,0.,-1.));
#25229=DIRECTION('ref_axis',(1.,0.,0.));
#25230=DIRECTION('center_axis',(0.,0.,1.));
#25231=DIRECTION('ref_axis',(1.,0.,0.));
#25232=DIRECTION('',(0.707106781186545,8.6595605623549E-17,-0.70710678118655));
#25233=DIRECTION('center_axis',(0.,0.,-1.));
#25234=DIRECTION('ref_axis',(1.,0.,0.));
#25235=DIRECTION('',(0.707106781186548,-8.65956056235493E-17,0.707106781186548));
#25236=DIRECTION('center_axis',(0.,0.,1.));
#25237=DIRECTION('ref_axis',(1.,0.,0.));
#25238=DIRECTION('center_axis',(0.,0.,1.));
#25239=DIRECTION('ref_axis',(1.,0.,0.));
#25240=DIRECTION('',(0.,0.,1.));
#25241=DIRECTION('center_axis',(0.,0.,-1.));
#25242=DIRECTION('ref_axis',(1.,0.,0.));
#25243=DIRECTION('center_axis',(0.,0.,1.));
#25244=DIRECTION('ref_axis',(1.,0.,0.));
#25245=DIRECTION('',(0.707106781186548,8.65956056235493E-17,-0.707106781186547));
#25246=DIRECTION('center_axis',(0.,0.,-1.));
#25247=DIRECTION('ref_axis',(1.,0.,0.));
#25248=DIRECTION('',(0.707106781186547,-8.65956056235493E-17,0.707106781186547));
#25249=DIRECTION('center_axis',(0.,0.,1.));
#25250=DIRECTION('ref_axis',(1.,0.,0.));
#25251=DIRECTION('center_axis',(0.,0.,1.));
#25252=DIRECTION('ref_axis',(1.,0.,0.));
#25253=DIRECTION('',(0.,0.,1.));
#25254=DIRECTION('center_axis',(0.,0.,-1.));
#25255=DIRECTION('ref_axis',(1.,0.,0.));
#25256=DIRECTION('center_axis',(0.,0.,1.));
#25257=DIRECTION('ref_axis',(1.,0.,0.));
#25258=DIRECTION('',(0.707106781186548,8.65956056235493E-17,-0.707106781186547));
#25259=DIRECTION('center_axis',(0.,0.,-1.));
#25260=DIRECTION('ref_axis',(1.,0.,0.));
#25261=DIRECTION('',(0.707106781186547,-8.65956056235493E-17,0.707106781186547));
#25262=DIRECTION('center_axis',(0.,0.,1.));
#25263=DIRECTION('ref_axis',(1.,0.,0.));
#25264=DIRECTION('center_axis',(0.,0.,1.));
#25265=DIRECTION('ref_axis',(1.,0.,0.));
#25266=DIRECTION('',(0.,0.,1.));
#25267=DIRECTION('center_axis',(0.,0.,-1.));
#25268=DIRECTION('ref_axis',(1.,0.,0.));
#25269=DIRECTION('center_axis',(0.,0.,1.));
#25270=DIRECTION('ref_axis',(1.,0.,0.));
#25271=DIRECTION('',(0.707106781186548,8.65956056235493E-17,-0.707106781186547));
#25272=DIRECTION('center_axis',(0.,0.,-1.));
#25273=DIRECTION('ref_axis',(1.,0.,0.));
#25274=DIRECTION('',(0.707106781186548,-8.65956056235493E-17,0.707106781186548));
#25275=DIRECTION('center_axis',(0.,0.,1.));
#25276=DIRECTION('ref_axis',(1.,0.,0.));
#25277=DIRECTION('center_axis',(0.,0.,1.));
#25278=DIRECTION('ref_axis',(1.,0.,0.));
#25279=DIRECTION('',(0.,0.,1.));
#25280=DIRECTION('center_axis',(0.,0.,-1.));
#25281=DIRECTION('ref_axis',(1.,0.,0.));
#25282=DIRECTION('center_axis',(0.,0.,1.));
#25283=DIRECTION('ref_axis',(1.,0.,0.));
#25284=DIRECTION('',(0.707106781186548,8.65956056235493E-17,-0.707106781186547));
#25285=DIRECTION('center_axis',(6.12323399573677E-17,0.,1.));
#25286=DIRECTION('ref_axis',(1.,0.,0.));
#25287=DIRECTION('center_axis',(1.22464679914735E-16,-1.,0.));
#25288=DIRECTION('ref_axis',(-1.,-1.22464679914735E-16,0.));
#25289=DIRECTION('center_axis',(0.,0.,1.));
#25290=DIRECTION('ref_axis',(1.,0.,0.));
#25291=DIRECTION('center_axis',(0.,0.,1.));
#25292=DIRECTION('ref_axis',(1.,0.,0.));
#25293=DIRECTION('',(0.707106781186549,8.65956056235496E-17,-0.707106781186546));
#25294=DIRECTION('center_axis',(0.,0.,1.));
#25295=DIRECTION('ref_axis',(1.,0.,0.));
#25296=DIRECTION('center_axis',(0.,0.,1.));
#25297=DIRECTION('ref_axis',(1.,0.,0.));
#25298=DIRECTION('',(0.,0.,-1.));
#25299=DIRECTION('center_axis',(0.,0.,-1.));
#25300=DIRECTION('ref_axis',(1.,0.,0.));
#25301=DIRECTION('',(-0.707106781186549,-8.65956056235496E-17,-0.707106781186546));
#30692=CARTESIAN_POINT('',(0.,0.,0.));
#30693=CARTESIAN_POINT('Origin',(2.02684561068023,-1.70072540437507,-0.28));
#30694=CARTESIAN_POINT('',(1.37684561068023,-1.70072540437507,-0.295));
#30695=CARTESIAN_POINT('Origin',(2.02684561068023,-1.70072540437507,-0.295));
#30696=CARTESIAN_POINT('',(1.40684561068023,-1.70072540437507,-0.265));
#30697=CARTESIAN_POINT('',(1.39184561068023,-1.70072540437507,-0.28));
#30698=CARTESIAN_POINT('Origin',(2.02684561068023,-1.70072540437507,-0.265));
#30699=CARTESIAN_POINT('Origin',(2.02684561068023,-1.70072540437507,-0.295));
#30700=CARTESIAN_POINT('',(1.40684561068023,-1.70072540437507,-0.025));
#30701=CARTESIAN_POINT('',(1.40684561068023,-1.70072540437507,-0.295));
#30702=CARTESIAN_POINT('Origin',(2.02684561068023,-1.70072540437507,-0.025));
#30703=CARTESIAN_POINT('Origin',(3.4,0.,-0.295));
#30704=CARTESIAN_POINT('',(-3.4,-4.163799117101E-16,-0.295));
#30705=CARTESIAN_POINT('Origin',(0.,0.,-0.295));
#30706=CARTESIAN_POINT('',(-3.13629421039049,0.904937086210529,-0.295));
#30707=CARTESIAN_POINT('Origin',(-2.48629421039049,0.904937086210529,-0.295));
#30708=CARTESIAN_POINT('',(1.99585903453311,7.96020419445779E-17,-0.295));
#30709=CARTESIAN_POINT('Origin',(2.64585903453311,0.,-0.295));
#30710=CARTESIAN_POINT('',(-3.13629421039049,-0.904937086210529,-0.295));
#30711=CARTESIAN_POINT('Origin',(-2.48629421039049,-0.904937086210529,-0.295));
#30712=CARTESIAN_POINT('',(-0.190551400289742,2.6056624905856,-0.295));
#30713=CARTESIAN_POINT('Origin',(0.459448599710258,2.6056624905856,-0.295));
#30714=CARTESIAN_POINT('',(-1.57765648986083,-1.93207197046211E-16,-0.295));
#30715=CARTESIAN_POINT('Origin',(0.,0.,-0.295));
#30716=CARTESIAN_POINT('',(-0.190551400289743,-2.6056624905856,-0.295));
#30717=CARTESIAN_POINT('Origin',(0.459448599710257,-2.6056624905856,-0.295));
#30718=CARTESIAN_POINT('',(-1.97292951726656,-2.29138113873824,-0.295));
#30719=CARTESIAN_POINT('Origin',(-1.32292951726656,-2.29138113873824,-0.295));
#30720=CARTESIAN_POINT('',(1.37684561068023,1.70072540437507,-0.295));
#30721=CARTESIAN_POINT('Origin',(2.02684561068023,1.70072540437507,-0.295));
#30722=CARTESIAN_POINT('',(-1.97292951726655,2.29138113873824,-0.295));
#30723=CARTESIAN_POINT('Origin',(-1.32292951726655,2.29138113873824,-0.295));
#30724=CARTESIAN_POINT('Origin',(2.02684561068023,-1.70072540437507,-0.01));
#30725=CARTESIAN_POINT('',(1.37684561068023,-1.70072540437507,0.005));
#30726=CARTESIAN_POINT('Origin',(2.02684561068023,-1.70072540437507,0.005));
#30727=CARTESIAN_POINT('',(1.39184561068023,-1.70072540437507,-0.01));
#30728=CARTESIAN_POINT('Origin',(1.60499221181911,0.,0.005));
#30729=CARTESIAN_POINT('',(-3.4,-4.163799117101E-16,0.00499999999999989));
#30730=CARTESIAN_POINT('Origin',(0.,0.,0.005));
#30731=CARTESIAN_POINT('',(-3.13629421039049,0.904937086210529,0.005));
#30732=CARTESIAN_POINT('Origin',(-2.48629421039049,0.904937086210529,0.005));
#30733=CARTESIAN_POINT('',(1.99585903453311,-7.96020419445779E-17,0.005));
#30734=CARTESIAN_POINT('Origin',(2.64585903453311,0.,0.005));
#30735=CARTESIAN_POINT('',(-3.13629421039049,-0.904937086210529,0.005));
#30736=CARTESIAN_POINT('Origin',(-2.48629421039049,-0.904937086210529,0.005));
#30737=CARTESIAN_POINT('',(-0.190551400289742,2.6056624905856,0.005));
#30738=CARTESIAN_POINT('Origin',(0.459448599710258,2.6056624905856,0.005));
#30739=CARTESIAN_POINT('',(-1.60499221181911,-1.9655485748607E-16,0.005));
#30740=CARTESIAN_POINT('Origin',(0.,0.,0.005));
#30741=CARTESIAN_POINT('',(-0.190551400289743,-2.6056624905856,0.005));
#30742=CARTESIAN_POINT('Origin',(0.459448599710257,-2.6056624905856,0.005));
#30743=CARTESIAN_POINT('',(-1.97292951726656,-2.29138113873824,0.005));
#30744=CARTESIAN_POINT('Origin',(-1.32292951726656,-2.29138113873824,0.005));
#30745=CARTESIAN_POINT('',(1.37684561068023,1.70072540437507,0.005));
#30746=CARTESIAN_POINT('Origin',(2.02684561068023,1.70072540437507,0.005));
#30747=CARTESIAN_POINT('',(-1.97292951726655,2.29138113873824,0.005));
#30748=CARTESIAN_POINT('Origin',(-1.32292951726655,2.29138113873824,0.005));
#30749=CARTESIAN_POINT('Origin',(-2.48629421039049,0.904937086210529,-0.28));
#30750=CARTESIAN_POINT('',(-3.10629421039049,0.904937086210529,-0.265));
#30751=CARTESIAN_POINT('',(-3.12129421039049,0.904937086210529,-0.28));
#30752=CARTESIAN_POINT('Origin',(-2.48629421039049,0.904937086210529,-0.265));
#30753=CARTESIAN_POINT('Origin',(-2.48629421039049,0.904937086210529,-0.295));
#30754=CARTESIAN_POINT('',(-3.10629421039049,0.904937086210529,-0.025));
#30755=CARTESIAN_POINT('',(-3.10629421039049,0.904937086210529,-0.295));
#30756=CARTESIAN_POINT('Origin',(-2.48629421039049,0.904937086210529,-0.025));
#30757=CARTESIAN_POINT('Origin',(-2.48629421039049,0.904937086210529,-0.01));
#30758=CARTESIAN_POINT('',(-3.12129421039049,0.904937086210529,-0.01));
#30759=CARTESIAN_POINT('Origin',(-1.32292951726655,2.29138113873824,-0.28));
#30760=CARTESIAN_POINT('',(-1.94292951726655,2.29138113873824,-0.265));
#30761=CARTESIAN_POINT('',(-1.95792951726655,2.29138113873824,-0.28));
#30762=CARTESIAN_POINT('Origin',(-1.32292951726655,2.29138113873824,-0.265));
#30763=CARTESIAN_POINT('Origin',(-1.32292951726655,2.29138113873824,-0.295));
#30764=CARTESIAN_POINT('',(-1.94292951726655,2.29138113873824,-0.025));
#30765=CARTESIAN_POINT('',(-1.94292951726655,2.29138113873824,-0.295));
#30766=CARTESIAN_POINT('Origin',(-1.32292951726655,2.29138113873824,-0.025));
#30767=CARTESIAN_POINT('Origin',(-1.32292951726655,2.29138113873824,-0.01));
#30768=CARTESIAN_POINT('',(-1.95792951726655,2.29138113873824,-0.01));
#30769=CARTESIAN_POINT('Origin',(2.64585903453311,0.,-0.28));
#30770=CARTESIAN_POINT('',(2.02585903453311,-7.59281015471359E-17,-0.265));
#30771=CARTESIAN_POINT('',(2.01085903453311,7.77650717458569E-17,-0.28));
#30772=CARTESIAN_POINT('Origin',(2.64585903453311,0.,-0.265));
#30773=CARTESIAN_POINT('Origin',(2.64585903453311,0.,-0.295));
#30774=CARTESIAN_POINT('',(2.02585903453311,7.59281015471359E-17,-0.025));
#30775=CARTESIAN_POINT('',(2.02585903453311,-7.59281015471359E-17,-0.295));
#30776=CARTESIAN_POINT('Origin',(2.64585903453311,0.,-0.025));
#30777=CARTESIAN_POINT('Origin',(2.64585903453311,0.,-0.01));
#30778=CARTESIAN_POINT('',(2.01085903453311,-7.77650717458569E-17,-0.01));
#30779=CARTESIAN_POINT('Origin',(2.02684561068023,1.70072540437507,-0.28));
#30780=CARTESIAN_POINT('',(1.40684561068023,1.70072540437507,-0.265));
#30781=CARTESIAN_POINT('',(1.39184561068023,1.70072540437507,-0.28));
#30782=CARTESIAN_POINT('Origin',(2.02684561068023,1.70072540437507,-0.265));
#30783=CARTESIAN_POINT('Origin',(2.02684561068023,1.70072540437507,-0.295));
#30784=CARTESIAN_POINT('',(1.40684561068023,1.70072540437507,-0.025));
#30785=CARTESIAN_POINT('',(1.40684561068023,1.70072540437507,-0.295));
#30786=CARTESIAN_POINT('Origin',(2.02684561068023,1.70072540437507,-0.025));
#30787=CARTESIAN_POINT('Origin',(2.02684561068023,1.70072540437507,-0.01));
#30788=CARTESIAN_POINT('',(1.39184561068023,1.70072540437507,-0.01));
#30789=CARTESIAN_POINT('Origin',(-2.48629421039049,-0.904937086210529,-0.28));
#30790=CARTESIAN_POINT('',(-3.10629421039049,-0.904937086210529,-0.265));
#30791=CARTESIAN_POINT('',(-3.12129421039049,-0.904937086210529,-0.28));
#30792=CARTESIAN_POINT('Origin',(-2.48629421039049,-0.904937086210529,-0.265));
#30793=CARTESIAN_POINT('Origin',(-2.48629421039049,-0.904937086210529,-0.295));
#30794=CARTESIAN_POINT('',(-3.10629421039049,-0.904937086210529,-0.025));
#30795=CARTESIAN_POINT('',(-3.10629421039049,-0.904937086210529,-0.295));
#30796=CARTESIAN_POINT('Origin',(-2.48629421039049,-0.904937086210529,-0.025));
#30797=CARTESIAN_POINT('Origin',(-2.48629421039049,-0.904937086210529,-0.01));
#30798=CARTESIAN_POINT('',(-3.12129421039049,-0.904937086210529,-0.01));
#30799=CARTESIAN_POINT('Origin',(-1.32292951726656,-2.29138113873824,-0.28));
#30800=CARTESIAN_POINT('',(-1.94292951726656,-2.29138113873824,-0.265));
#30801=CARTESIAN_POINT('',(-1.95792951726656,-2.29138113873824,-0.28));
#30802=CARTESIAN_POINT('Origin',(-1.32292951726656,-2.29138113873824,-0.265));
#30803=CARTESIAN_POINT('Origin',(-1.32292951726656,-2.29138113873824,-0.295));
#30804=CARTESIAN_POINT('',(-1.94292951726656,-2.29138113873824,-0.025));
#30805=CARTESIAN_POINT('',(-1.94292951726656,-2.29138113873824,-0.295));
#30806=CARTESIAN_POINT('Origin',(-1.32292951726656,-2.29138113873824,-0.025));
#30807=CARTESIAN_POINT('Origin',(-1.32292951726656,-2.29138113873824,-0.01));
#30808=CARTESIAN_POINT('',(-1.95792951726656,-2.29138113873824,-0.01));
#30809=CARTESIAN_POINT('Origin',(0.459448599710258,2.6056624905856,-0.28));
#30810=CARTESIAN_POINT('',(-0.160551400289742,2.6056624905856,-0.265));
#30811=CARTESIAN_POINT('',(-0.175551400289742,2.6056624905856,-0.28));
#30812=CARTESIAN_POINT('Origin',(0.459448599710258,2.6056624905856,-0.265));
#30813=CARTESIAN_POINT('Origin',(0.459448599710258,2.6056624905856,-0.295));
#30814=CARTESIAN_POINT('',(-0.160551400289742,2.6056624905856,-0.025));
#30815=CARTESIAN_POINT('',(-0.160551400289742,2.6056624905856,-0.295));
#30816=CARTESIAN_POINT('Origin',(0.459448599710258,2.6056624905856,-0.025));
#30817=CARTESIAN_POINT('Origin',(0.459448599710258,2.6056624905856,-0.01));
#30818=CARTESIAN_POINT('',(-0.175551400289742,2.6056624905856,-0.01));
#30819=CARTESIAN_POINT('Origin',(0.459448599710257,-2.6056624905856,-0.28));
#30820=CARTESIAN_POINT('',(-0.160551400289743,-2.6056624905856,-0.265));
#30821=CARTESIAN_POINT('',(-0.175551400289743,-2.6056624905856,-0.28));
#30822=CARTESIAN_POINT('Origin',(0.459448599710257,-2.6056624905856,-0.265));
#30823=CARTESIAN_POINT('Origin',(0.459448599710257,-2.6056624905856,-0.295));
#30824=CARTESIAN_POINT('',(-0.160551400289743,-2.6056624905856,-0.025));
#30825=CARTESIAN_POINT('',(-0.160551400289743,-2.6056624905856,-0.295));
#30826=CARTESIAN_POINT('Origin',(0.459448599710257,-2.6056624905856,-0.025));
#30827=CARTESIAN_POINT('Origin',(0.459448599710257,-2.6056624905856,-0.01));
#30828=CARTESIAN_POINT('',(-0.175551400289743,-2.6056624905856,-0.01));
#30829=CARTESIAN_POINT('Origin',(-1.77635683940025E-15,0.,8.32667268468867E-17));
#30830=CARTESIAN_POINT('Origin',(-1.77635683940025E-15,0.,8.32667268468867E-17));
#30831=CARTESIAN_POINT('Origin',(0.,0.,-0.27));
#30832=CARTESIAN_POINT('',(-3.45,-4.22503145705837E-16,-0.245));
#30833=CARTESIAN_POINT('Origin',(0.,0.,-0.245));
#30834=CARTESIAN_POINT('',(-3.425,-4.19441528707968E-16,-0.27));
#30835=CARTESIAN_POINT('Origin',(0.,0.,-0.145));
#30836=CARTESIAN_POINT('',(-3.45,-4.22503145705837E-16,-0.045));
#30837=CARTESIAN_POINT('Origin',(0.,0.,-0.045));
#30838=CARTESIAN_POINT('',(-3.45,-4.22503145705837E-16,-0.145));
#30839=CARTESIAN_POINT('Origin',(0.,0.,-0.02));
#30840=CARTESIAN_POINT('',(-3.425,-4.19441528707968E-16,-0.02));
#59162=UNCERTAINTY_MEASURE_WITH_UNIT(LENGTH_MEASURE(0.001),#59205,
'DISTANCE_ACCURACY_VALUE',
'Maximum model space distance between geometric entities at asserted c
onnectivities');
#59182=UNCERTAINTY_MEASURE_WITH_UNIT(LENGTH_MEASURE(0.001),#59205,
'DISTANCE_ACCURACY_VALUE',
'Maximum model space distance between geometric entities at asserted c
onnectivities');
#59184=(
GEOMETRIC_REPRESENTATION_CONTEXT(3)
GLOBAL_UNCERTAINTY_ASSIGNED_CONTEXT((#59162))
GLOBAL_UNIT_ASSIGNED_CONTEXT((#59205,#59207,#59208))
REPRESENTATION_CONTEXT('','3D')
);
#59204=(
GEOMETRIC_REPRESENTATION_CONTEXT(3)
GLOBAL_UNCERTAINTY_ASSIGNED_CONTEXT((#59182))
GLOBAL_UNIT_ASSIGNED_CONTEXT((#59205,#59207,#59208))
REPRESENTATION_CONTEXT('','3D')
);
#59205=(
LENGTH_UNIT()
NAMED_UNIT(*)
SI_UNIT(.CENTI.,.METRE.)
);
#59207=(
NAMED_UNIT(*)
PLANE_ANGLE_UNIT()
SI_UNIT($,.RADIAN.)
);
#59208=(
NAMED_UNIT(*)
SI_UNIT($,.STERADIAN.)
SOLID_ANGLE_UNIT()
);
#59210=SHAPE_DEFINITION_REPRESENTATION(#59231,#59297);
#59231=PRODUCT_DEFINITION_SHAPE('',$,#59319);
#59297=SHAPE_REPRESENTATION('',(#23046),#59184);
#59317=PRODUCT_DEFINITION_CONTEXT('part definition',#59382,'design');
#59319=PRODUCT_DEFINITION('2026-10-23-00-47-18-389',
'08_Slipper_Retainer_Plate',#59340,#59317);
#59340=PRODUCT_DEFINITION_FORMATION('',$,#59385);
#59382=APPLICATION_CONTEXT(
'Core Data for Automotive Mechanical Design Process');
#59383=PRODUCT_CONTEXT('part definition',#59382,'mechanical');
#59385=PRODUCT('2026-10-23-00-47-18-389','08_Slipper_Retainer_Plate',$,
(#59383));
#59573=COLOUR_RGB('Sky Blue',0.24,0.69,0.87);
#59574=FILL_AREA_STYLE_COLOUR('',#59573);
#59575=FILL_AREA_STYLE('',(#59574));
#59576=SURFACE_STYLE_FILL_AREA(#59575);
#59577=SURFACE_SIDE_STYLE('',(#59576));
#59578=SURFACE_STYLE_USAGE(.BOTH.,#59577);
#59579=PRESENTATION_STYLE_ASSIGNMENT((#59578));
ENDSEC;
END-ISO-10303-21;
